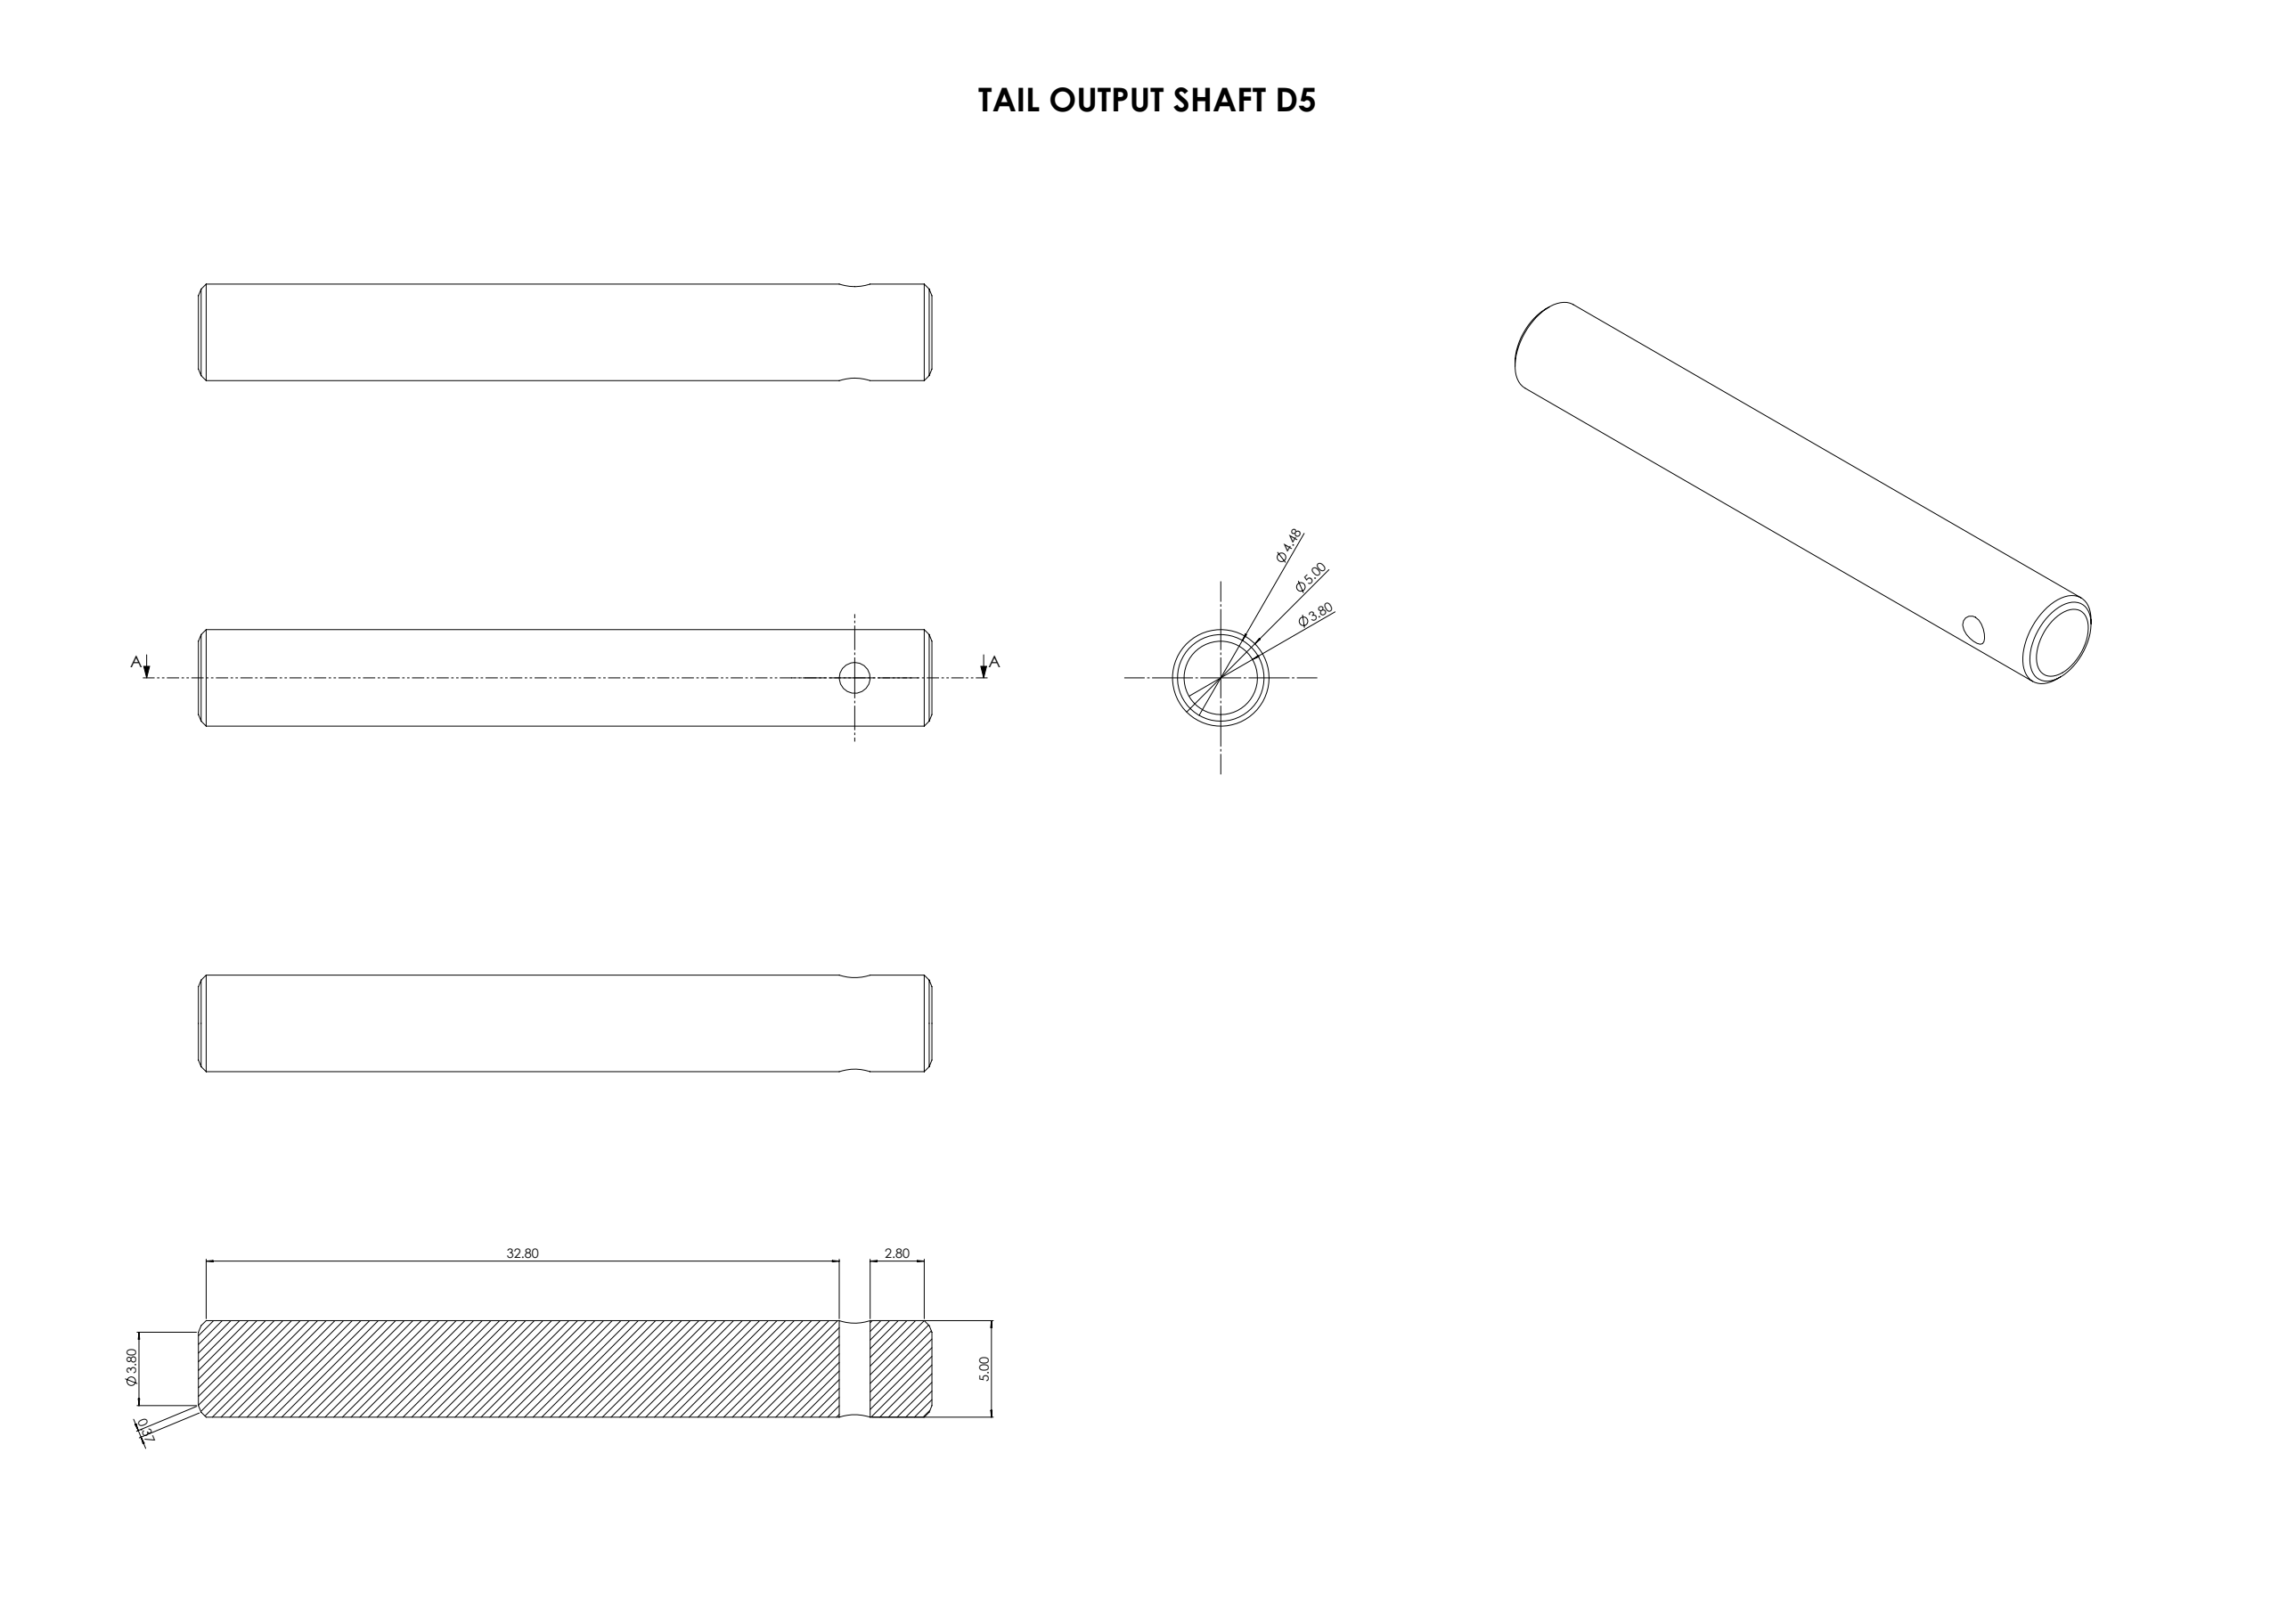
ISO-10303-21;
HEADER;
/* Generated by software containing ST-Developer
 * from STEP Tools, Inc. (www.steptools.com) 
 */

FILE_DESCRIPTION(
/* description */ (''),
/* implementation_level */ '2;1');

FILE_NAME(
/* name */ '12_Tail_Output_Shaft_D5.step',
/* time_stamp */ '2026-10-25T01:35:35-07:00',
/* author */ (''),
/* organization */ (''),
/* preprocessor_version */ 'ST-DEVELOPER v20.2',
/* originating_system */ 'Autodesk Translation Framework v15.15.0.0',
/* authorisation */ '');

FILE_SCHEMA (('AUTOMOTIVE_DESIGN { 1 0 10303 214 3 1 1 }'));
ENDSEC;

DATA;
#10=MECHANICAL_DESIGN_GEOMETRIC_PRESENTATION_REPRESENTATION('',(#267),#11430);
#160=B_SPLINE_CURVE_WITH_KNOTS('',3,(#9138,#9139,#9140,#9141,#9142,#9143,
#9144,#9145,#9146,#9147,#9148,#9149,#9150,#9151,#9152,#9153,#9154,#9155,
#9156,#9157,#9158,#9159,#9160,#9161,#9162,#9163),.UNSPECIFIED.,.F.,.F.,
(4,2,2,2,2,2,2,2,2,2,2,2,4),(0.,0.0303730235339956,0.0607460470679912,0.0911072107271434,
0.121468374386296,0.151829538045448,0.1821907017046,0.212563725238596,0.242936748772591,
0.273309772306587,0.303682795840582,0.334043959499734,0.364405123158887),
 .UNSPECIFIED.);
#161=B_SPLINE_CURVE_WITH_KNOTS('',3,(#9164,#9165,#9166,#9167,#9168,#9169,
#9170,#9171,#9172,#9173),.UNSPECIFIED.,.F.,.F.,(4,2,2,2,4),(0.364405123158887,
0.394766286818039,0.425127450477191,0.455500474011187,0.485873497545182),
 .UNSPECIFIED.);
#162=B_SPLINE_CURVE_WITH_KNOTS('',3,(#9177,#9178,#9179,#9180,#9181,#9182,
#9183,#9184,#9185,#9186),.UNSPECIFIED.,.F.,.F.,(4,2,2,2,4),(0.,0.0303730235339955,
0.060746047067991,0.0911072107271433,0.121468374386295),.UNSPECIFIED.);
#163=B_SPLINE_CURVE_WITH_KNOTS('',3,(#9187,#9188,#9189,#9190,#9191,#9192,
#9193,#9194,#9195,#9196,#9197,#9198,#9199,#9200,#9201,#9202,#9203,#9204,
#9205,#9206,#9207,#9208,#9209,#9210,#9211,#9212),.UNSPECIFIED.,.F.,.F.,
(4,2,2,2,2,2,2,2,2,2,2,2,4),(0.121468374386295,0.151829538045448,0.1821907017046,
0.212563725238595,0.242936748772591,0.273309772306587,0.303682795840582,
0.334043959499734,0.364405123158887,0.394766286818039,0.425127450477191,
0.455500474011187,0.485873497545182),.UNSPECIFIED.);
#243=SHAPE_REPRESENTATION_RELATIONSHIP('SRR','None',#11486,#255);
#255=ADVANCED_BREP_SHAPE_REPRESENTATION('',(#279),#11425);
#267=STYLED_ITEM('',(#11609),#279);
#279=MANIFOLD_SOLID_BREP('Body1',#4468);
#310=FACE_BOUND('',#992,.T.);
#311=FACE_BOUND('',#993,.T.);
#393=PLANE('',#4904);
#394=PLANE('',#4909);
#484=CYLINDRICAL_SURFACE('',#4912,0.800000000000001);
#485=CYLINDRICAL_SURFACE('',#4913,2.5);
#690=FACE_OUTER_BOUND('',#984,.T.);
#691=FACE_OUTER_BOUND('',#985,.T.);
#692=FACE_OUTER_BOUND('',#986,.T.);
#693=FACE_OUTER_BOUND('',#987,.T.);
#694=FACE_OUTER_BOUND('',#988,.T.);
#695=FACE_OUTER_BOUND('',#989,.T.);
#696=FACE_OUTER_BOUND('',#990,.T.);
#697=FACE_OUTER_BOUND('',#991,.T.);
#984=EDGE_LOOP('',(#3639,#3640,#3641,#3642,#3643));
#985=EDGE_LOOP('',(#3644,#3645,#3646,#3647,#3648));
#986=EDGE_LOOP('',(#3649));
#987=EDGE_LOOP('',(#3650,#3651,#3652,#3653,#3654));
#988=EDGE_LOOP('',(#3655));
#989=EDGE_LOOP('',(#3656,#3657,#3658,#3659,#3660));
#990=EDGE_LOOP('',(#3661,#3662,#3663,#3664,#3665,#3666));
#991=EDGE_LOOP('',(#3667,#3668,#3669,#3670));
#992=EDGE_LOOP('',(#3671,#3672));
#993=EDGE_LOOP('',(#3673,#3674));
#1265=LINE('',#9113,#1555);
#1266=LINE('',#9119,#1556);
#1267=LINE('',#9128,#1557);
#1268=LINE('',#9134,#1558);
#1269=LINE('',#9175,#1559);
#1270=LINE('',#9214,#1560);
#1555=VECTOR('',#5835,2.07071067811866);
#1556=VECTOR('',#5842,2.3);
#1557=VECTOR('',#5853,2.07071067811866);
#1558=VECTOR('',#5862,2.3);
#1559=VECTOR('',#5865,0.800000000000001);
#1560=VECTOR('',#5868,2.5);
#1804=CIRCLE('',#4899,1.9);
#1805=CIRCLE('',#4900,2.24142135623731);
#1806=CIRCLE('',#4901,2.24142135623731);
#1807=CIRCLE('',#4903,2.5);
#1808=CIRCLE('',#4906,2.24142135623731);
#1809=CIRCLE('',#4907,2.24142135623731);
#1810=CIRCLE('',#4908,1.9);
#1811=CIRCLE('',#4911,2.5);
#2103=VERTEX_POINT('',#9110);
#2104=VERTEX_POINT('',#9112);
#2105=VERTEX_POINT('',#9114);
#2106=VERTEX_POINT('',#9118);
#2107=VERTEX_POINT('',#9123);
#2108=VERTEX_POINT('',#9124);
#2109=VERTEX_POINT('',#9127);
#2110=VERTEX_POINT('',#9132);
#2111=VERTEX_POINT('',#9136);
#2112=VERTEX_POINT('',#9137);
#2113=VERTEX_POINT('',#9174);
#2114=VERTEX_POINT('',#9176);
#2637=EDGE_CURVE('',#2103,#2103,#1804,.T.);
#2638=EDGE_CURVE('',#2103,#2104,#1265,.T.);
#2639=EDGE_CURVE('',#2104,#2105,#1805,.T.);
#2640=EDGE_CURVE('',#2105,#2104,#1806,.T.);
#2641=EDGE_CURVE('',#2105,#2106,#1266,.T.);
#2642=EDGE_CURVE('',#2106,#2106,#1807,.T.);
#2643=EDGE_CURVE('',#2107,#2108,#1808,.T.);
#2644=EDGE_CURVE('',#2108,#2107,#1809,.T.);
#2645=EDGE_CURVE('',#2107,#2109,#1267,.T.);
#2646=EDGE_CURVE('',#2109,#2109,#1810,.T.);
#2647=EDGE_CURVE('',#2110,#2110,#1811,.T.);
#2648=EDGE_CURVE('',#2110,#2108,#1268,.T.);
#2649=EDGE_CURVE('',#2111,#2112,#160,.T.);
#2650=EDGE_CURVE('',#2112,#2111,#161,.T.);
#2651=EDGE_CURVE('',#2112,#2113,#1269,.T.);
#2652=EDGE_CURVE('',#2114,#2113,#162,.T.);
#2653=EDGE_CURVE('',#2113,#2114,#163,.T.);
#2654=EDGE_CURVE('',#2106,#2110,#1270,.T.);
#3639=ORIENTED_EDGE('',*,*,#2637,.T.);
#3640=ORIENTED_EDGE('',*,*,#2638,.T.);
#3641=ORIENTED_EDGE('',*,*,#2639,.T.);
#3642=ORIENTED_EDGE('',*,*,#2640,.T.);
#3643=ORIENTED_EDGE('',*,*,#2638,.F.);
#3644=ORIENTED_EDGE('',*,*,#2639,.F.);
#3645=ORIENTED_EDGE('',*,*,#2640,.F.);
#3646=ORIENTED_EDGE('',*,*,#2641,.T.);
#3647=ORIENTED_EDGE('',*,*,#2642,.T.);
#3648=ORIENTED_EDGE('',*,*,#2641,.F.);
#3649=ORIENTED_EDGE('',*,*,#2637,.F.);
#3650=ORIENTED_EDGE('',*,*,#2643,.T.);
#3651=ORIENTED_EDGE('',*,*,#2644,.T.);
#3652=ORIENTED_EDGE('',*,*,#2645,.T.);
#3653=ORIENTED_EDGE('',*,*,#2646,.T.);
#3654=ORIENTED_EDGE('',*,*,#2645,.F.);
#3655=ORIENTED_EDGE('',*,*,#2646,.F.);
#3656=ORIENTED_EDGE('',*,*,#2647,.F.);
#3657=ORIENTED_EDGE('',*,*,#2648,.T.);
#3658=ORIENTED_EDGE('',*,*,#2643,.F.);
#3659=ORIENTED_EDGE('',*,*,#2644,.F.);
#3660=ORIENTED_EDGE('',*,*,#2648,.F.);
#3661=ORIENTED_EDGE('',*,*,#2649,.F.);
#3662=ORIENTED_EDGE('',*,*,#2650,.F.);
#3663=ORIENTED_EDGE('',*,*,#2651,.T.);
#3664=ORIENTED_EDGE('',*,*,#2652,.F.);
#3665=ORIENTED_EDGE('',*,*,#2653,.F.);
#3666=ORIENTED_EDGE('',*,*,#2651,.F.);
#3667=ORIENTED_EDGE('',*,*,#2642,.F.);
#3668=ORIENTED_EDGE('',*,*,#2654,.T.);
#3669=ORIENTED_EDGE('',*,*,#2647,.T.);
#3670=ORIENTED_EDGE('',*,*,#2654,.F.);
#3671=ORIENTED_EDGE('',*,*,#2652,.T.);
#3672=ORIENTED_EDGE('',*,*,#2653,.T.);
#3673=ORIENTED_EDGE('',*,*,#2649,.T.);
#3674=ORIENTED_EDGE('',*,*,#2650,.T.);
#4171=CONICAL_SURFACE('',#4898,2.07071067811866,1.17809724509617);
#4172=CONICAL_SURFACE('',#4902,2.3,0.785398163397453);
#4173=CONICAL_SURFACE('',#4905,2.07071067811866,1.17809724509617);
#4174=CONICAL_SURFACE('',#4910,2.3,0.785398163397448);
#4357=ADVANCED_FACE('',(#690),#4171,.T.);
#4358=ADVANCED_FACE('',(#691),#4172,.T.);
#4359=ADVANCED_FACE('',(#692),#393,.T.);
#4360=ADVANCED_FACE('',(#693),#4173,.T.);
#4361=ADVANCED_FACE('',(#694),#394,.T.);
#4362=ADVANCED_FACE('',(#695),#4174,.T.);
#4363=ADVANCED_FACE('',(#696),#484,.F.);
#4364=ADVANCED_FACE('',(#697,#310,#311),#485,.T.);
#4468=CLOSED_SHELL('',(#4357,#4358,#4359,#4360,#4361,#4362,#4363,#4364));
#4897=AXIS2_PLACEMENT_3D('',#9108,#5829,#5830);
#4898=AXIS2_PLACEMENT_3D('',#9109,#5831,#5832);
#4899=AXIS2_PLACEMENT_3D('',#9111,#5833,#5834);
#4900=AXIS2_PLACEMENT_3D('',#9115,#5836,#5837);
#4901=AXIS2_PLACEMENT_3D('',#9116,#5838,#5839);
#4902=AXIS2_PLACEMENT_3D('',#9117,#5840,#5841);
#4903=AXIS2_PLACEMENT_3D('',#9120,#5843,#5844);
#4904=AXIS2_PLACEMENT_3D('',#9121,#5845,#5846);
#4905=AXIS2_PLACEMENT_3D('',#9122,#5847,#5848);
#4906=AXIS2_PLACEMENT_3D('',#9125,#5849,#5850);
#4907=AXIS2_PLACEMENT_3D('',#9126,#5851,#5852);
#4908=AXIS2_PLACEMENT_3D('',#9129,#5854,#5855);
#4909=AXIS2_PLACEMENT_3D('',#9130,#5856,#5857);
#4910=AXIS2_PLACEMENT_3D('',#9131,#5858,#5859);
#4911=AXIS2_PLACEMENT_3D('',#9133,#5860,#5861);
#4912=AXIS2_PLACEMENT_3D('',#9135,#5863,#5864);
#4913=AXIS2_PLACEMENT_3D('',#9213,#5866,#5867);
#5829=DIRECTION('axis',(0.,0.,1.));
#5830=DIRECTION('refdir',(1.,0.,0.));
#5831=DIRECTION('center_axis',(-1.,0.,-9.70486199004632E-16));
#5832=DIRECTION('ref_axis',(0.,-1.,-3.31401861020786E-17));
#5833=DIRECTION('center_axis',(-1.,0.,0.));
#5834=DIRECTION('ref_axis',(0.,-1.,0.));
#5835=DIRECTION('',(-0.382683432365091,0.923879532511287,-2.27628838825947E-16));
#5836=DIRECTION('center_axis',(1.,0.,0.));
#5837=DIRECTION('ref_axis',(0.,-1.,-6.12323399573677E-17));
#5838=DIRECTION('center_axis',(1.,0.,0.));
#5839=DIRECTION('ref_axis',(0.,-1.,-6.12323399573677E-17));
#5840=DIRECTION('center_axis',(-1.,0.,0.));
#5841=DIRECTION('ref_axis',(0.,1.,0.));
#5842=DIRECTION('',(-0.707106781186544,-0.707106781186551,-8.65956056235497E-17));
#5843=DIRECTION('center_axis',(1.,0.,0.));
#5844=DIRECTION('ref_axis',(0.,0.,-1.));
#5845=DIRECTION('center_axis',(1.,0.,0.));
#5846=DIRECTION('ref_axis',(0.,0.,-1.));
#5847=DIRECTION('center_axis',(1.,0.,-9.70486199004632E-16));
#5848=DIRECTION('ref_axis',(0.,-1.,-3.31401861020786E-17));
#5849=DIRECTION('center_axis',(-1.,0.,0.));
#5850=DIRECTION('ref_axis',(0.,-1.,-6.12323399573677E-17));
#5851=DIRECTION('center_axis',(-1.,0.,0.));
#5852=DIRECTION('ref_axis',(0.,-1.,-6.12323399573677E-17));
#5853=DIRECTION('',(-0.382683432365091,-0.923879532511287,2.27628838825947E-16));
#5854=DIRECTION('center_axis',(1.,0.,0.));
#5855=DIRECTION('ref_axis',(0.,-1.,0.));
#5856=DIRECTION('center_axis',(-1.,0.,0.));
#5857=DIRECTION('ref_axis',(0.,0.,1.));
#5858=DIRECTION('center_axis',(1.,0.,0.));
#5859=DIRECTION('ref_axis',(0.,1.,0.));
#5860=DIRECTION('center_axis',(1.,0.,0.));
#5861=DIRECTION('ref_axis',(0.,0.,-1.));
#5862=DIRECTION('',(-0.707106781186548,0.707106781186547,8.65956056235493E-17));
#5863=DIRECTION('center_axis',(0.,0.,-1.));
#5864=DIRECTION('ref_axis',(1.,0.,0.));
#5865=DIRECTION('',(0.,0.,-1.));
#5866=DIRECTION('center_axis',(1.,0.,0.));
#5867=DIRECTION('ref_axis',(0.,1.,0.));
#5868=DIRECTION('',(-1.,0.,0.));
#9108=CARTESIAN_POINT('',(0.,0.,0.));
#9109=CARTESIAN_POINT('Origin',(23.9292893218813,0.,-6.86237372364135E-17));
#9110=CARTESIAN_POINT('',(24.,1.9,-2.32682891837997E-16));
#9111=CARTESIAN_POINT('Origin',(24.,0.,0.));
#9112=CARTESIAN_POINT('',(23.8585786437627,2.24142135623731,2.74494948945654E-16));
#9113=CARTESIAN_POINT('',(23.9292893218813,2.07071067811866,2.53588920391826E-16));
#9114=CARTESIAN_POINT('',(23.8585786437627,-2.24142135623731,-2.74494948945654E-16));
#9115=CARTESIAN_POINT('Origin',(23.8585786437627,0.,-1.37247474472827E-16));
#9116=CARTESIAN_POINT('Origin',(23.8585786437627,0.,-1.37247474472827E-16));
#9117=CARTESIAN_POINT('Origin',(23.8,0.,0.));
#9118=CARTESIAN_POINT('',(23.6,-2.5,-3.06161699786838E-16));
#9119=CARTESIAN_POINT('',(23.8,-2.3,-2.81668763803891E-16));
#9120=CARTESIAN_POINT('Origin',(23.6,0.,0.));
#9121=CARTESIAN_POINT('Origin',(24.,0.,0.));
#9122=CARTESIAN_POINT('Origin',(-13.9292893218813,0.,-6.86237372364135E-17));
#9123=CARTESIAN_POINT('',(-13.8585786437627,2.24142135623731,-2.74494948945654E-16));
#9124=CARTESIAN_POINT('',(-13.8585786437627,-2.24142135623731,-2.74494948945654E-16));
#9125=CARTESIAN_POINT('Origin',(-13.8585786437627,0.,-1.37247474472827E-16));
#9126=CARTESIAN_POINT('Origin',(-13.8585786437627,0.,-1.37247474472827E-16));
#9127=CARTESIAN_POINT('',(-14.,1.9,2.32682891837997E-16));
#9128=CARTESIAN_POINT('',(-13.9292893218813,2.07071067811866,2.53588920391826E-16));
#9129=CARTESIAN_POINT('Origin',(-14.,0.,0.));
#9130=CARTESIAN_POINT('Origin',(-14.,2.1,0.));
#9131=CARTESIAN_POINT('Origin',(-13.8,0.,0.));
#9132=CARTESIAN_POINT('',(-13.6,-2.5,-3.06161699786838E-16));
#9133=CARTESIAN_POINT('Origin',(-13.6,0.,0.));
#9134=CARTESIAN_POINT('',(-13.8,-2.3,-2.81668763803891E-16));
#9135=CARTESIAN_POINT('Origin',(20.,0.,3.));
#9136=CARTESIAN_POINT('',(20.,0.800000000000001,2.3685438564654));
#9137=CARTESIAN_POINT('',(19.2,9.79717439317883E-17,2.5));
#9138=CARTESIAN_POINT('Ctrl Pts',(20.,0.800000000000001,2.3685438564654));
#9139=CARTESIAN_POINT('Ctrl Pts',(20.10124341178,0.800000000000001,2.3685438564654));
#9140=CARTESIAN_POINT('Ctrl Pts',(20.2087021071075,0.779619973172144,2.37571629748165));
#9141=CARTESIAN_POINT('Ctrl Pts',(20.4055671254356,0.697767352464298,2.40103225043771));
#9142=CARTESIAN_POINT('Ctrl Pts',(20.4950422069344,0.63632864296403,2.41874877205569));
#9143=CARTESIAN_POINT('Ctrl Pts',(20.6363010586268,0.495069791271689,2.45156308488026));
#9144=CARTESIAN_POINT('Ctrl Pts',(20.697761056251,0.405583630634407,2.46887493070887));
#9145=CARTESIAN_POINT('Ctrl Pts',(20.7796294856729,0.208677866314441,2.49324989776594));
#9146=CARTESIAN_POINT('Ctrl Pts',(20.8,0.101203878863841,2.5));
#9147=CARTESIAN_POINT('Ctrl Pts',(20.8,-0.101203878863841,2.5));
#9148=CARTESIAN_POINT('Ctrl Pts',(20.7796294856729,-0.208677866314441,2.49324989776594));
#9149=CARTESIAN_POINT('Ctrl Pts',(20.697761056251,-0.405583630634407,2.46887493070887));
#9150=CARTESIAN_POINT('Ctrl Pts',(20.6363010586268,-0.495069791271689,2.45156308488026));
#9151=CARTESIAN_POINT('Ctrl Pts',(20.4950422069344,-0.63632864296403,2.41874877205569));
#9152=CARTESIAN_POINT('Ctrl Pts',(20.4055671254356,-0.697767352464298,2.40103225043771));
#9153=CARTESIAN_POINT('Ctrl Pts',(20.2087021071075,-0.779619973172144,2.37571629748165));
#9154=CARTESIAN_POINT('Ctrl Pts',(20.10124341178,-0.800000000000001,2.3685438564654));
#9155=CARTESIAN_POINT('Ctrl Pts',(19.89875658822,-0.800000000000001,2.3685438564654));
#9156=CARTESIAN_POINT('Ctrl Pts',(19.7912978928925,-0.779619973172145,2.37571629748165));
#9157=CARTESIAN_POINT('Ctrl Pts',(19.5944328745644,-0.697767352464302,2.40103225043771));
#9158=CARTESIAN_POINT('Ctrl Pts',(19.5049577930656,-0.636328642964029,2.41874877205569));
#9159=CARTESIAN_POINT('Ctrl Pts',(19.3636989413732,-0.495069791271689,2.45156308488026));
#9160=CARTESIAN_POINT('Ctrl Pts',(19.302238943749,-0.405583630634409,2.46887493070887));
#9161=CARTESIAN_POINT('Ctrl Pts',(19.2203705143271,-0.208677866314441,2.49324989776594));
#9162=CARTESIAN_POINT('Ctrl Pts',(19.2,-0.101203878863841,2.5));
#9163=CARTESIAN_POINT('Ctrl Pts',(19.2,-6.93889390390723E-17,2.5));
#9164=CARTESIAN_POINT('Ctrl Pts',(19.2,-1.21430643318376E-16,2.5));
#9165=CARTESIAN_POINT('Ctrl Pts',(19.2,0.101203878863841,2.5));
#9166=CARTESIAN_POINT('Ctrl Pts',(19.2203705143271,0.208677866314441,2.49324989776594));
#9167=CARTESIAN_POINT('Ctrl Pts',(19.302238943749,0.405583630634408,2.46887493070887));
#9168=CARTESIAN_POINT('Ctrl Pts',(19.3636989413732,0.495069791271689,2.45156308488026));
#9169=CARTESIAN_POINT('Ctrl Pts',(19.5049577930656,0.636328642964029,2.41874877205569));
#9170=CARTESIAN_POINT('Ctrl Pts',(19.5944328745644,0.697767352464302,2.40103225043771));
#9171=CARTESIAN_POINT('Ctrl Pts',(19.7912978928925,0.779619973172145,2.37571629748165));
#9172=CARTESIAN_POINT('Ctrl Pts',(19.89875658822,0.800000000000001,2.3685438564654));
#9173=CARTESIAN_POINT('Ctrl Pts',(20.,0.800000000000001,2.3685438564654));
#9174=CARTESIAN_POINT('',(19.2,9.79717439317883E-17,-2.5));
#9175=CARTESIAN_POINT('',(19.2,9.79717439317883E-17,3.));
#9176=CARTESIAN_POINT('',(20.,0.800000000000001,-2.3685438564654));
#9177=CARTESIAN_POINT('Ctrl Pts',(20.,0.800000000000001,-2.3685438564654));
#9178=CARTESIAN_POINT('Ctrl Pts',(19.89875658822,0.800000000000001,-2.3685438564654));
#9179=CARTESIAN_POINT('Ctrl Pts',(19.7912978928925,0.779619973172145,-2.37571629748165));
#9180=CARTESIAN_POINT('Ctrl Pts',(19.5944328745644,0.697767352464302,-2.40103225043771));
#9181=CARTESIAN_POINT('Ctrl Pts',(19.5049577930656,0.636328642964029,-2.41874877205569));
#9182=CARTESIAN_POINT('Ctrl Pts',(19.3636989413732,0.495069791271689,-2.45156308488026));
#9183=CARTESIAN_POINT('Ctrl Pts',(19.302238943749,0.405583630634408,-2.46887493070887));
#9184=CARTESIAN_POINT('Ctrl Pts',(19.2203705143271,0.208677866314441,-2.49324989776594));
#9185=CARTESIAN_POINT('Ctrl Pts',(19.2,0.101203878863841,-2.5));
#9186=CARTESIAN_POINT('Ctrl Pts',(19.2,-1.73472347597681E-17,-2.5));
#9187=CARTESIAN_POINT('Ctrl Pts',(19.2,-2.16840434497101E-16,-2.5));
#9188=CARTESIAN_POINT('Ctrl Pts',(19.2,-0.101203878863841,-2.5));
#9189=CARTESIAN_POINT('Ctrl Pts',(19.2203705143271,-0.208677866314441,-2.49324989776594));
#9190=CARTESIAN_POINT('Ctrl Pts',(19.302238943749,-0.405583630634408,-2.46887493070887));
#9191=CARTESIAN_POINT('Ctrl Pts',(19.3636989413732,-0.495069791271689,-2.45156308488026));
#9192=CARTESIAN_POINT('Ctrl Pts',(19.5049577930656,-0.636328642964029,-2.41874877205569));
#9193=CARTESIAN_POINT('Ctrl Pts',(19.5944328745644,-0.697767352464302,-2.40103225043771));
#9194=CARTESIAN_POINT('Ctrl Pts',(19.7912978928925,-0.779619973172145,-2.37571629748165));
#9195=CARTESIAN_POINT('Ctrl Pts',(19.89875658822,-0.800000000000001,-2.3685438564654));
#9196=CARTESIAN_POINT('Ctrl Pts',(20.10124341178,-0.800000000000001,-2.3685438564654));
#9197=CARTESIAN_POINT('Ctrl Pts',(20.2087021071075,-0.779619973172144,-2.37571629748165));
#9198=CARTESIAN_POINT('Ctrl Pts',(20.4055671254356,-0.697767352464298,-2.40103225043771));
#9199=CARTESIAN_POINT('Ctrl Pts',(20.4950422069344,-0.63632864296403,-2.41874877205569));
#9200=CARTESIAN_POINT('Ctrl Pts',(20.6363010586268,-0.495069791271689,-2.45156308488026));
#9201=CARTESIAN_POINT('Ctrl Pts',(20.697761056251,-0.405583630634407,-2.46887493070887));
#9202=CARTESIAN_POINT('Ctrl Pts',(20.7796294856729,-0.208677866314441,-2.49324989776594));
#9203=CARTESIAN_POINT('Ctrl Pts',(20.8,-0.101203878863841,-2.5));
#9204=CARTESIAN_POINT('Ctrl Pts',(20.8,0.101203878863841,-2.5));
#9205=CARTESIAN_POINT('Ctrl Pts',(20.7796294856729,0.208677866314441,-2.49324989776594));
#9206=CARTESIAN_POINT('Ctrl Pts',(20.697761056251,0.405583630634407,-2.46887493070887));
#9207=CARTESIAN_POINT('Ctrl Pts',(20.6363010586268,0.495069791271689,-2.45156308488026));
#9208=CARTESIAN_POINT('Ctrl Pts',(20.4950422069344,0.63632864296403,-2.41874877205569));
#9209=CARTESIAN_POINT('Ctrl Pts',(20.4055671254356,0.697767352464298,-2.40103225043771));
#9210=CARTESIAN_POINT('Ctrl Pts',(20.2087021071075,0.779619973172144,-2.37571629748165));
#9211=CARTESIAN_POINT('Ctrl Pts',(20.10124341178,0.8,-2.3685438564654));
#9212=CARTESIAN_POINT('Ctrl Pts',(20.,0.8,-2.3685438564654));
#9213=CARTESIAN_POINT('Origin',(5.,0.,0.));
#9214=CARTESIAN_POINT('',(5.,-2.5,-3.06161699786838E-16));
#11411=UNCERTAINTY_MEASURE_WITH_UNIT(LENGTH_MEASURE(0.01),#11431,
'DISTANCE_ACCURACY_VALUE',
'Maximum model space distance between geometric entities at asserted c
onnectivities');
#11416=UNCERTAINTY_MEASURE_WITH_UNIT(LENGTH_MEASURE(0.01),#11431,
'DISTANCE_ACCURACY_VALUE',
'Maximum model space distance between geometric entities at asserted c
onnectivities');
#11425=(
GEOMETRIC_REPRESENTATION_CONTEXT(3)
GLOBAL_UNCERTAINTY_ASSIGNED_CONTEXT((#11411))
GLOBAL_UNIT_ASSIGNED_CONTEXT((#11431,#11433,#11434))
REPRESENTATION_CONTEXT('','3D')
);
#11430=(
GEOMETRIC_REPRESENTATION_CONTEXT(3)
GLOBAL_UNCERTAINTY_ASSIGNED_CONTEXT((#11416))
GLOBAL_UNIT_ASSIGNED_CONTEXT((#11431,#11433,#11434))
REPRESENTATION_CONTEXT('','3D')
);
#11431=(
LENGTH_UNIT()
NAMED_UNIT(*)
SI_UNIT(.MILLI.,.METRE.)
);
#11433=(
NAMED_UNIT(*)
PLANE_ANGLE_UNIT()
SI_UNIT($,.RADIAN.)
);
#11434=(
NAMED_UNIT(*)
SI_UNIT($,.STERADIAN.)
SOLID_ANGLE_UNIT()
);
#11443=SHAPE_DEFINITION_REPRESENTATION(#11456,#11486);
#11456=PRODUCT_DEFINITION_SHAPE('',$,#11500);
#11486=SHAPE_REPRESENTATION('',(#4897),#11425);
#11491=PRODUCT_DEFINITION_CONTEXT('part definition',#11532,'design');
#11500=PRODUCT_DEFINITION('2026-10-25-00-55-41-884',
'12_Tail_Output_Shaft_D5',#11513,#11491);
#11513=PRODUCT_DEFINITION_FORMATION('',$,#11542);
#11532=APPLICATION_CONTEXT(
'Core Data for Automotive Mechanical Design Process');
#11533=PRODUCT_CONTEXT('part definition',#11532,'mechanical');
#11542=PRODUCT('2026-10-25-00-55-41-884','12_Tail_Output_Shaft_D5',$,(#11533));
#11603=COLOUR_RGB('Grey',0.48,0.52,0.57);
#11604=FILL_AREA_STYLE_COLOUR('',#11603);
#11605=FILL_AREA_STYLE('',(#11604));
#11606=SURFACE_STYLE_FILL_AREA(#11605);
#11607=SURFACE_SIDE_STYLE('',(#11606));
#11608=SURFACE_STYLE_USAGE(.BOTH.,#11607);
#11609=PRESENTATION_STYLE_ASSIGNMENT((#11608));
ENDSEC;
END-ISO-10303-21;
